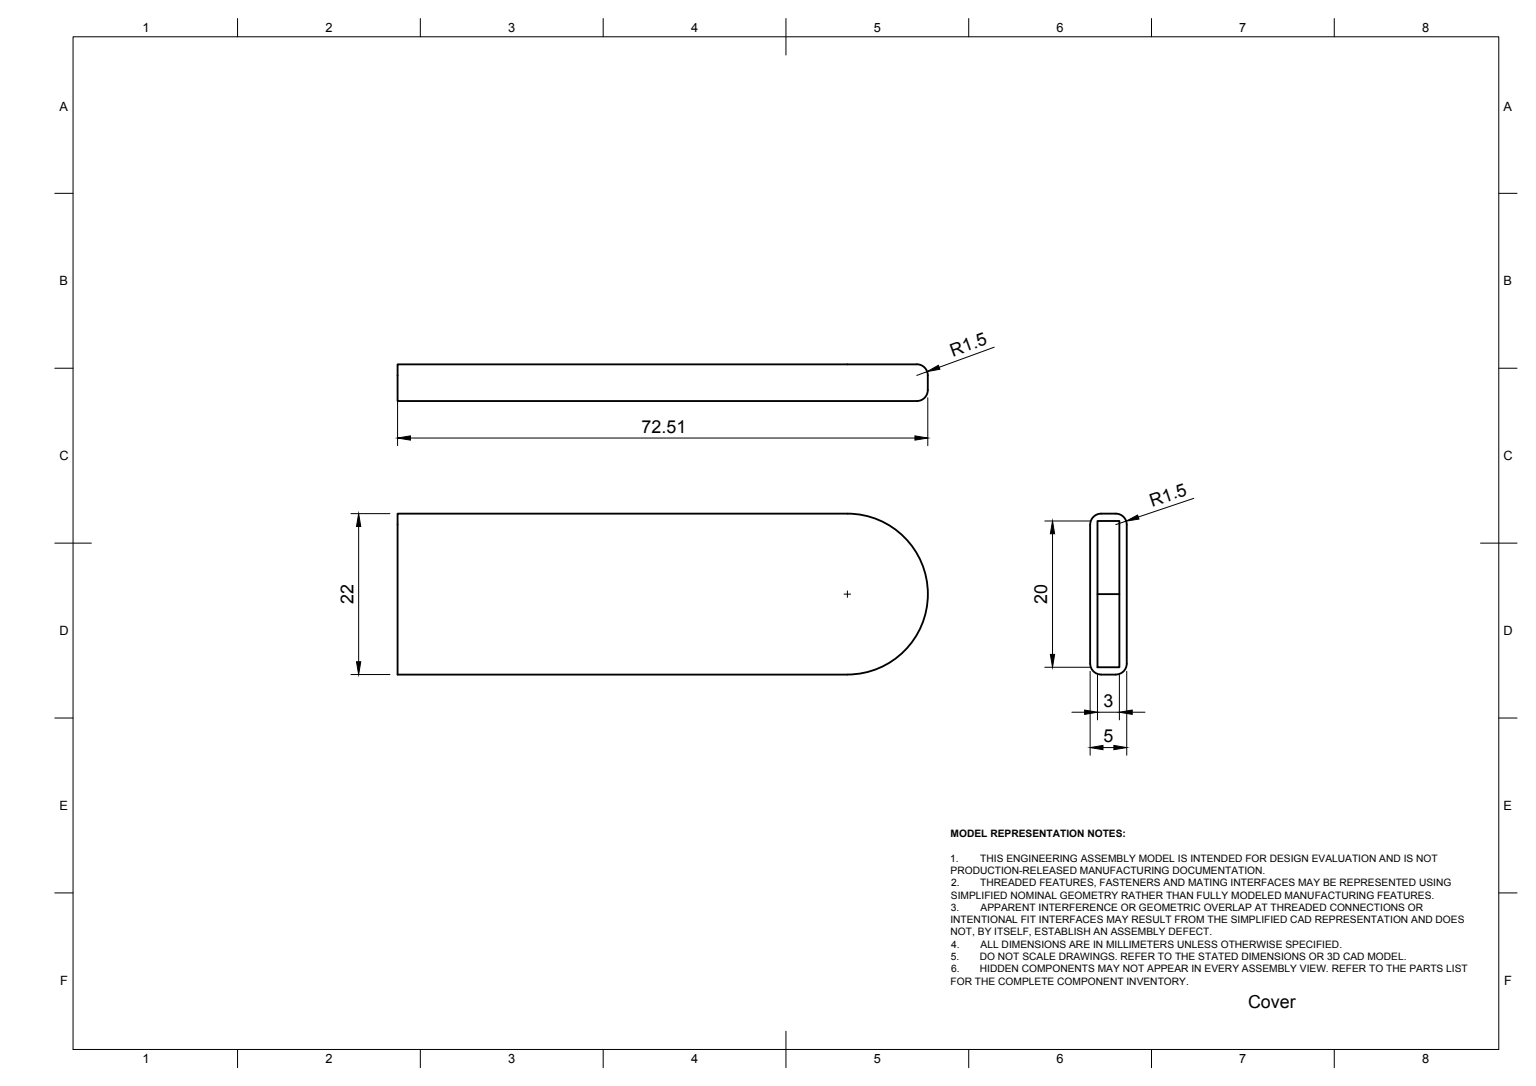
ISO-10303-21;
HEADER;
/* Generated by software containing ST-Developer
 * from STEP Tools, Inc. (www.steptools.com) 
 */

FILE_DESCRIPTION(
/* description */ (''),
/* implementation_level */ '2;1');

FILE_NAME(
/* name */ 'Cover.step',
/* time_stamp */ '2026-10-06T12:47:13-07:00',
/* author */ (''),
/* organization */ (''),
/* preprocessor_version */ 'ST-DEVELOPER v20.2',
/* originating_system */ 'Autodesk Translation Framework v15.15.0.0',
/* authorisation */ '');

FILE_SCHEMA (('AUTOMOTIVE_DESIGN { 1 0 10303 214 3 1 1 }'));
ENDSEC;

DATA;
#10=MECHANICAL_DESIGN_GEOMETRIC_PRESENTATION_REPRESENTATION('',(#68),#42667);
#50=SHAPE_REPRESENTATION_RELATIONSHIP('SRR','None',#42703,#59);
#59=ADVANCED_BREP_SHAPE_REPRESENTATION('',(#77),#42659);
#68=STYLED_ITEM('',(#42756),#77);
#77=MANIFOLD_SOLID_BREP('Body1',#4033);
#387=FACE_BOUND('',#884,.T.);
#403=CYLINDRICAL_SURFACE('',#4197,1.5);
#404=CYLINDRICAL_SURFACE('',#4204,1.5);
#405=CYLINDRICAL_SURFACE('',#4207,11.);
#406=CYLINDRICAL_SURFACE('',#4210,1.5);
#407=CYLINDRICAL_SURFACE('',#4216,1.5);
#408=CYLINDRICAL_SURFACE('',#4220,30.);
#409=CYLINDRICAL_SURFACE('',#4224,30.);
#503=TOROIDAL_SURFACE('',#4200,9.5,1.5);
#504=TOROIDAL_SURFACE('',#4213,9.5,1.5);
#544=CIRCLE('',#4198,1.5);
#545=CIRCLE('',#4199,1.5);
#546=CIRCLE('',#4201,1.5);
#547=CIRCLE('',#4202,11.);
#548=CIRCLE('',#4203,9.5);
#549=CIRCLE('',#4205,1.5);
#550=CIRCLE('',#4208,11.);
#551=CIRCLE('',#4211,1.5);
#552=CIRCLE('',#4212,1.5);
#553=CIRCLE('',#4214,1.5);
#554=CIRCLE('',#4215,9.5);
#555=CIRCLE('',#4217,1.5);
#556=CIRCLE('',#4221,30.);
#557=CIRCLE('',#4222,30.);
#558=CIRCLE('',#4225,30.);
#559=CIRCLE('',#4226,30.);
#667=FACE_OUTER_BOUND('',#873,.T.);
#668=FACE_OUTER_BOUND('',#874,.T.);
#669=FACE_OUTER_BOUND('',#875,.T.);
#670=FACE_OUTER_BOUND('',#876,.T.);
#671=FACE_OUTER_BOUND('',#877,.T.);
#672=FACE_OUTER_BOUND('',#878,.T.);
#673=FACE_OUTER_BOUND('',#879,.T.);
#674=FACE_OUTER_BOUND('',#880,.T.);
#675=FACE_OUTER_BOUND('',#881,.T.);
#676=FACE_OUTER_BOUND('',#882,.T.);
#677=FACE_OUTER_BOUND('',#883,.T.);
#678=FACE_OUTER_BOUND('',#885,.T.);
#679=FACE_OUTER_BOUND('',#886,.T.);
#680=FACE_OUTER_BOUND('',#887,.T.);
#681=FACE_OUTER_BOUND('',#888,.T.);
#682=FACE_OUTER_BOUND('',#889,.T.);
#683=FACE_OUTER_BOUND('',#890,.T.);
#684=FACE_OUTER_BOUND('',#891,.T.);
#873=EDGE_LOOP('',(#2660,#2661,#2662,#2663));
#874=EDGE_LOOP('',(#2664,#2665,#2666,#2667));
#875=EDGE_LOOP('',(#2668,#2669,#2670,#2671));
#876=EDGE_LOOP('',(#2672,#2673,#2674,#2675));
#877=EDGE_LOOP('',(#2676,#2677,#2678,#2679));
#878=EDGE_LOOP('',(#2680,#2681,#2682,#2683));
#879=EDGE_LOOP('',(#2684,#2685,#2686,#2687));
#880=EDGE_LOOP('',(#2688,#2689,#2690,#2691));
#881=EDGE_LOOP('',(#2692,#2693,#2694,#2695));
#882=EDGE_LOOP('',(#2696,#2697,#2698,#2699));
#883=EDGE_LOOP('',(#2700,#2701,#2702,#2703,#2704,#2705,#2706,#2707));
#884=EDGE_LOOP('',(#2708,#2709,#2710,#2711));
#885=EDGE_LOOP('',(#2712,#2713,#2714,#2715));
#886=EDGE_LOOP('',(#2716,#2717,#2718,#2719));
#887=EDGE_LOOP('',(#2720,#2721,#2722,#2723));
#888=EDGE_LOOP('',(#2724,#2725,#2726,#2727,#2728));
#889=EDGE_LOOP('',(#2729,#2730,#2731,#2732));
#890=EDGE_LOOP('',(#2733,#2734,#2735,#2736,#2737));
#891=EDGE_LOOP('',(#2738,#2739,#2740,#2741));
#1082=LINE('',#5866,#1295);
#1083=LINE('',#5869,#1296);
#1084=LINE('',#5880,#1297);
#1085=LINE('',#5881,#1298);
#1086=LINE('',#5884,#1299);
#1087=LINE('',#5886,#1300);
#1088=LINE('',#5887,#1301);
#1089=LINE('',#5890,#1302);
#1090=LINE('',#5894,#1303);
#1091=LINE('',#5895,#1304);
#1092=LINE('',#5900,#1305);
#1093=LINE('',#5909,#1306);
#1094=LINE('',#5911,#1307);
#1095=LINE('',#5913,#1308);
#1096=LINE('',#5916,#1309);
#1097=LINE('',#5918,#1310);
#1098=LINE('',#5920,#1311);
#1099=LINE('',#5921,#1312);
#1100=LINE('',#5927,#1313);
#1101=LINE('',#5930,#1314);
#1102=LINE('',#5932,#1315);
#1103=LINE('',#5933,#1316);
#1104=LINE('',#5938,#1317);
#1105=LINE('',#5941,#1318);
#1106=LINE('',#5943,#1319);
#1295=VECTOR('',#4615,10.);
#1296=VECTOR('',#4618,10.);
#1297=VECTOR('',#4631,10.);
#1298=VECTOR('',#4632,10.);
#1299=VECTOR('',#4635,10.);
#1300=VECTOR('',#4636,10.);
#1301=VECTOR('',#4637,10.);
#1302=VECTOR('',#4640,10.);
#1303=VECTOR('',#4645,10.);
#1304=VECTOR('',#4646,10.);
#1305=VECTOR('',#4651,10.);
#1306=VECTOR('',#4664,10.);
#1307=VECTOR('',#4667,10.);
#1308=VECTOR('',#4670,10.);
#1309=VECTOR('',#4671,10.);
#1310=VECTOR('',#4672,10.);
#1311=VECTOR('',#4673,10.);
#1312=VECTOR('',#4674,10.);
#1313=VECTOR('',#4679,10.);
#1314=VECTOR('',#4682,30.);
#1315=VECTOR('',#4685,10.);
#1316=VECTOR('',#4686,10.);
#1317=VECTOR('',#4691,30.);
#1318=VECTOR('',#4696,10.);
#1319=VECTOR('',#4699,10.);
#1516=VERTEX_POINT('',#5862);
#1517=VERTEX_POINT('',#5863);
#1518=VERTEX_POINT('',#5865);
#1519=VERTEX_POINT('',#5867);
#1520=VERTEX_POINT('',#5871);
#1521=VERTEX_POINT('',#5872);
#1522=VERTEX_POINT('',#5877);
#1523=VERTEX_POINT('',#5878);
#1524=VERTEX_POINT('',#5883);
#1525=VERTEX_POINT('',#5885);
#1526=VERTEX_POINT('',#5889);
#1527=VERTEX_POINT('',#5893);
#1528=VERTEX_POINT('',#5897);
#1529=VERTEX_POINT('',#5899);
#1530=VERTEX_POINT('',#5903);
#1531=VERTEX_POINT('',#5907);
#1532=VERTEX_POINT('',#5914);
#1533=VERTEX_POINT('',#5915);
#1534=VERTEX_POINT('',#5917);
#1535=VERTEX_POINT('',#5919);
#1536=VERTEX_POINT('',#5923);
#1537=VERTEX_POINT('',#5924);
#1538=VERTEX_POINT('',#5926);
#1539=VERTEX_POINT('',#5928);
#1540=VERTEX_POINT('',#5935);
#1541=VERTEX_POINT('',#5937);
#1981=EDGE_CURVE('',#1516,#1517,#544,.T.);
#1982=EDGE_CURVE('',#1517,#1518,#1082,.T.);
#1983=EDGE_CURVE('',#1518,#1519,#545,.T.);
#1984=EDGE_CURVE('',#1519,#1516,#1083,.T.);
#1985=EDGE_CURVE('',#1520,#1521,#546,.T.);
#1986=EDGE_CURVE('',#1521,#1519,#547,.T.);
#1987=EDGE_CURVE('',#1518,#1520,#548,.T.);
#1988=EDGE_CURVE('',#1522,#1523,#549,.T.);
#1989=EDGE_CURVE('',#1523,#1521,#1084,.T.);
#1990=EDGE_CURVE('',#1520,#1522,#1085,.T.);
#1991=EDGE_CURVE('',#1519,#1524,#1086,.T.);
#1992=EDGE_CURVE('',#1525,#1524,#1087,.T.);
#1993=EDGE_CURVE('',#1516,#1525,#1088,.T.);
#1994=EDGE_CURVE('',#1521,#1526,#1089,.T.);
#1995=EDGE_CURVE('',#1524,#1526,#550,.T.);
#1996=EDGE_CURVE('',#1523,#1527,#1090,.T.);
#1997=EDGE_CURVE('',#1526,#1527,#1091,.T.);
#1998=EDGE_CURVE('',#1527,#1528,#551,.T.);
#1999=EDGE_CURVE('',#1528,#1529,#1092,.T.);
#2000=EDGE_CURVE('',#1529,#1526,#552,.T.);
#2001=EDGE_CURVE('',#1530,#1524,#553,.T.);
#2002=EDGE_CURVE('',#1529,#1530,#554,.T.);
#2003=EDGE_CURVE('',#1531,#1525,#555,.T.);
#2004=EDGE_CURVE('',#1530,#1531,#1093,.T.);
#2005=EDGE_CURVE('',#1531,#1528,#1094,.T.);
#2006=EDGE_CURVE('',#1517,#1522,#1095,.T.);
#2007=EDGE_CURVE('',#1532,#1533,#1096,.T.);
#2008=EDGE_CURVE('',#1534,#1533,#1097,.T.);
#2009=EDGE_CURVE('',#1535,#1534,#1098,.T.);
#2010=EDGE_CURVE('',#1535,#1532,#1099,.T.);
#2011=EDGE_CURVE('',#1536,#1537,#556,.T.);
#2012=EDGE_CURVE('',#1537,#1538,#1100,.T.);
#2013=EDGE_CURVE('',#1538,#1539,#557,.T.);
#2014=EDGE_CURVE('',#1536,#1539,#1101,.T.);
#2015=EDGE_CURVE('',#1539,#1532,#1102,.T.);
#2016=EDGE_CURVE('',#1535,#1536,#1103,.T.);
#2017=EDGE_CURVE('',#1540,#1537,#558,.T.);
#2018=EDGE_CURVE('',#1540,#1541,#1104,.T.);
#2019=EDGE_CURVE('',#1538,#1541,#559,.T.);
#2020=EDGE_CURVE('',#1534,#1540,#1105,.T.);
#2021=EDGE_CURVE('',#1541,#1533,#1106,.T.);
#2660=ORIENTED_EDGE('',*,*,#1981,.T.);
#2661=ORIENTED_EDGE('',*,*,#1982,.T.);
#2662=ORIENTED_EDGE('',*,*,#1983,.T.);
#2663=ORIENTED_EDGE('',*,*,#1984,.T.);
#2664=ORIENTED_EDGE('',*,*,#1985,.T.);
#2665=ORIENTED_EDGE('',*,*,#1986,.T.);
#2666=ORIENTED_EDGE('',*,*,#1983,.F.);
#2667=ORIENTED_EDGE('',*,*,#1987,.T.);
#2668=ORIENTED_EDGE('',*,*,#1988,.T.);
#2669=ORIENTED_EDGE('',*,*,#1989,.T.);
#2670=ORIENTED_EDGE('',*,*,#1985,.F.);
#2671=ORIENTED_EDGE('',*,*,#1990,.T.);
#2672=ORIENTED_EDGE('',*,*,#1984,.F.);
#2673=ORIENTED_EDGE('',*,*,#1991,.T.);
#2674=ORIENTED_EDGE('',*,*,#1992,.F.);
#2675=ORIENTED_EDGE('',*,*,#1993,.F.);
#2676=ORIENTED_EDGE('',*,*,#1986,.F.);
#2677=ORIENTED_EDGE('',*,*,#1994,.T.);
#2678=ORIENTED_EDGE('',*,*,#1995,.F.);
#2679=ORIENTED_EDGE('',*,*,#1991,.F.);
#2680=ORIENTED_EDGE('',*,*,#1989,.F.);
#2681=ORIENTED_EDGE('',*,*,#1996,.T.);
#2682=ORIENTED_EDGE('',*,*,#1997,.F.);
#2683=ORIENTED_EDGE('',*,*,#1994,.F.);
#2684=ORIENTED_EDGE('',*,*,#1998,.T.);
#2685=ORIENTED_EDGE('',*,*,#1999,.T.);
#2686=ORIENTED_EDGE('',*,*,#2000,.T.);
#2687=ORIENTED_EDGE('',*,*,#1997,.T.);
#2688=ORIENTED_EDGE('',*,*,#2001,.T.);
#2689=ORIENTED_EDGE('',*,*,#1995,.T.);
#2690=ORIENTED_EDGE('',*,*,#2000,.F.);
#2691=ORIENTED_EDGE('',*,*,#2002,.T.);
#2692=ORIENTED_EDGE('',*,*,#2003,.T.);
#2693=ORIENTED_EDGE('',*,*,#1992,.T.);
#2694=ORIENTED_EDGE('',*,*,#2001,.F.);
#2695=ORIENTED_EDGE('',*,*,#2004,.T.);
#2696=ORIENTED_EDGE('',*,*,#2004,.F.);
#2697=ORIENTED_EDGE('',*,*,#2002,.F.);
#2698=ORIENTED_EDGE('',*,*,#1999,.F.);
#2699=ORIENTED_EDGE('',*,*,#2005,.F.);
#2700=ORIENTED_EDGE('',*,*,#1981,.F.);
#2701=ORIENTED_EDGE('',*,*,#1993,.T.);
#2702=ORIENTED_EDGE('',*,*,#2003,.F.);
#2703=ORIENTED_EDGE('',*,*,#2005,.T.);
#2704=ORIENTED_EDGE('',*,*,#1998,.F.);
#2705=ORIENTED_EDGE('',*,*,#1996,.F.);
#2706=ORIENTED_EDGE('',*,*,#1988,.F.);
#2707=ORIENTED_EDGE('',*,*,#2006,.F.);
#2708=ORIENTED_EDGE('',*,*,#2007,.T.);
#2709=ORIENTED_EDGE('',*,*,#2008,.F.);
#2710=ORIENTED_EDGE('',*,*,#2009,.F.);
#2711=ORIENTED_EDGE('',*,*,#2010,.T.);
#2712=ORIENTED_EDGE('',*,*,#2011,.T.);
#2713=ORIENTED_EDGE('',*,*,#2012,.T.);
#2714=ORIENTED_EDGE('',*,*,#2013,.T.);
#2715=ORIENTED_EDGE('',*,*,#2014,.F.);
#2716=ORIENTED_EDGE('',*,*,#2014,.T.);
#2717=ORIENTED_EDGE('',*,*,#2015,.T.);
#2718=ORIENTED_EDGE('',*,*,#2010,.F.);
#2719=ORIENTED_EDGE('',*,*,#2016,.T.);
#2720=ORIENTED_EDGE('',*,*,#2017,.F.);
#2721=ORIENTED_EDGE('',*,*,#2018,.T.);
#2722=ORIENTED_EDGE('',*,*,#2019,.F.);
#2723=ORIENTED_EDGE('',*,*,#2012,.F.);
#2724=ORIENTED_EDGE('',*,*,#2017,.T.);
#2725=ORIENTED_EDGE('',*,*,#2011,.F.);
#2726=ORIENTED_EDGE('',*,*,#2016,.F.);
#2727=ORIENTED_EDGE('',*,*,#2009,.T.);
#2728=ORIENTED_EDGE('',*,*,#2020,.T.);
#2729=ORIENTED_EDGE('',*,*,#2018,.F.);
#2730=ORIENTED_EDGE('',*,*,#2020,.F.);
#2731=ORIENTED_EDGE('',*,*,#2008,.T.);
#2732=ORIENTED_EDGE('',*,*,#2021,.F.);
#2733=ORIENTED_EDGE('',*,*,#2019,.T.);
#2734=ORIENTED_EDGE('',*,*,#2021,.T.);
#2735=ORIENTED_EDGE('',*,*,#2007,.F.);
#2736=ORIENTED_EDGE('',*,*,#2015,.F.);
#2737=ORIENTED_EDGE('',*,*,#2013,.F.);
#2738=ORIENTED_EDGE('',*,*,#1982,.F.);
#2739=ORIENTED_EDGE('',*,*,#2006,.T.);
#2740=ORIENTED_EDGE('',*,*,#1990,.F.);
#2741=ORIENTED_EDGE('',*,*,#1987,.F.);
#3788=PLANE('',#4206);
#3789=PLANE('',#4209);
#3790=PLANE('',#4218);
#3791=PLANE('',#4219);
#3792=PLANE('',#4223);
#3793=PLANE('',#4227);
#3794=PLANE('',#4228);
#3795=PLANE('',#4229);
#3796=PLANE('',#4230);
#3863=ADVANCED_FACE('',(#667),#403,.T.);
#3864=ADVANCED_FACE('',(#668),#503,.T.);
#3865=ADVANCED_FACE('',(#669),#404,.T.);
#3866=ADVANCED_FACE('',(#670),#3788,.F.);
#3867=ADVANCED_FACE('',(#671),#405,.T.);
#3868=ADVANCED_FACE('',(#672),#3789,.T.);
#3869=ADVANCED_FACE('',(#673),#406,.T.);
#3870=ADVANCED_FACE('',(#674),#504,.T.);
#3871=ADVANCED_FACE('',(#675),#407,.T.);
#3872=ADVANCED_FACE('',(#676),#3790,.T.);
#3873=ADVANCED_FACE('',(#677,#387),#3791,.T.);
#3874=ADVANCED_FACE('',(#678),#408,.F.);
#3875=ADVANCED_FACE('',(#679),#3792,.F.);
#3876=ADVANCED_FACE('',(#680),#409,.F.);
#3877=ADVANCED_FACE('',(#681),#3793,.T.);
#3878=ADVANCED_FACE('',(#682),#3794,.T.);
#3879=ADVANCED_FACE('',(#683),#3795,.T.);
#3880=ADVANCED_FACE('',(#684),#3796,.T.);
#4033=CLOSED_SHELL('',(#3863,#3864,#3865,#3866,#3867,#3868,#3869,#3870,
#3871,#3872,#3873,#3874,#3875,#3876,#3877,#3878,#3879,#3880));
#4196=AXIS2_PLACEMENT_3D('',#5860,#4609,#4610);
#4197=AXIS2_PLACEMENT_3D('',#5861,#4611,#4612);
#4198=AXIS2_PLACEMENT_3D('',#5864,#4613,#4614);
#4199=AXIS2_PLACEMENT_3D('',#5868,#4616,#4617);
#4200=AXIS2_PLACEMENT_3D('',#5870,#4619,#4620);
#4201=AXIS2_PLACEMENT_3D('',#5873,#4621,#4622);
#4202=AXIS2_PLACEMENT_3D('',#5874,#4623,#4624);
#4203=AXIS2_PLACEMENT_3D('',#5875,#4625,#4626);
#4204=AXIS2_PLACEMENT_3D('',#5876,#4627,#4628);
#4205=AXIS2_PLACEMENT_3D('',#5879,#4629,#4630);
#4206=AXIS2_PLACEMENT_3D('',#5882,#4633,#4634);
#4207=AXIS2_PLACEMENT_3D('',#5888,#4638,#4639);
#4208=AXIS2_PLACEMENT_3D('',#5891,#4641,#4642);
#4209=AXIS2_PLACEMENT_3D('',#5892,#4643,#4644);
#4210=AXIS2_PLACEMENT_3D('',#5896,#4647,#4648);
#4211=AXIS2_PLACEMENT_3D('',#5898,#4649,#4650);
#4212=AXIS2_PLACEMENT_3D('',#5901,#4652,#4653);
#4213=AXIS2_PLACEMENT_3D('',#5902,#4654,#4655);
#4214=AXIS2_PLACEMENT_3D('',#5904,#4656,#4657);
#4215=AXIS2_PLACEMENT_3D('',#5905,#4658,#4659);
#4216=AXIS2_PLACEMENT_3D('',#5906,#4660,#4661);
#4217=AXIS2_PLACEMENT_3D('',#5908,#4662,#4663);
#4218=AXIS2_PLACEMENT_3D('',#5910,#4665,#4666);
#4219=AXIS2_PLACEMENT_3D('',#5912,#4668,#4669);
#4220=AXIS2_PLACEMENT_3D('',#5922,#4675,#4676);
#4221=AXIS2_PLACEMENT_3D('',#5925,#4677,#4678);
#4222=AXIS2_PLACEMENT_3D('',#5929,#4680,#4681);
#4223=AXIS2_PLACEMENT_3D('',#5931,#4683,#4684);
#4224=AXIS2_PLACEMENT_3D('',#5934,#4687,#4688);
#4225=AXIS2_PLACEMENT_3D('',#5936,#4689,#4690);
#4226=AXIS2_PLACEMENT_3D('',#5939,#4692,#4693);
#4227=AXIS2_PLACEMENT_3D('',#5940,#4694,#4695);
#4228=AXIS2_PLACEMENT_3D('',#5942,#4697,#4698);
#4229=AXIS2_PLACEMENT_3D('',#5944,#4700,#4701);
#4230=AXIS2_PLACEMENT_3D('',#5945,#4702,#4703);
#4609=DIRECTION('axis',(0.,0.,1.));
#4610=DIRECTION('refdir',(1.,0.,0.));
#4611=DIRECTION('center_axis',(0.,1.,0.));
#4612=DIRECTION('ref_axis',(-0.707106781186547,0.,-0.707106781186548));
#4613=DIRECTION('center_axis',(0.,-1.,0.));
#4614=DIRECTION('ref_axis',(-0.707106781186547,0.,-0.707106781186548));
#4615=DIRECTION('',(0.,-1.,0.));
#4616=DIRECTION('center_axis',(0.,1.,0.));
#4617=DIRECTION('ref_axis',(0.,0.,-1.));
#4618=DIRECTION('',(0.,1.,0.));
#4619=DIRECTION('center_axis',(0.,0.,1.));
#4620=DIRECTION('ref_axis',(1.,0.,0.));
#4621=DIRECTION('center_axis',(0.,-1.,0.));
#4622=DIRECTION('ref_axis',(0.,0.,-1.));
#4623=DIRECTION('center_axis',(0.,0.,-1.));
#4624=DIRECTION('ref_axis',(1.00929365875014E-16,-1.,0.));
#4625=DIRECTION('center_axis',(0.,0.,1.));
#4626=DIRECTION('ref_axis',(1.00929365875014E-16,-1.,0.));
#4627=DIRECTION('center_axis',(0.,1.,0.));
#4628=DIRECTION('ref_axis',(0.707106781186547,0.,-0.707106781186548));
#4629=DIRECTION('center_axis',(0.,-1.,0.));
#4630=DIRECTION('ref_axis',(0.707106781186547,0.,-0.707106781186548));
#4631=DIRECTION('',(0.,-1.,0.));
#4632=DIRECTION('',(0.,1.,0.));
#4633=DIRECTION('center_axis',(1.,0.,0.));
#4634=DIRECTION('ref_axis',(0.,0.,-1.));
#4635=DIRECTION('',(0.,0.,1.));
#4636=DIRECTION('',(0.,-1.,0.));
#4637=DIRECTION('',(0.,0.,1.));
#4638=DIRECTION('center_axis',(0.,0.,-1.));
#4639=DIRECTION('ref_axis',(0.707106781186547,-0.707106781186548,0.));
#4640=DIRECTION('',(0.,0.,1.));
#4641=DIRECTION('center_axis',(0.,0.,1.));
#4642=DIRECTION('ref_axis',(-5.04646829375071E-16,-1.,0.));
#4643=DIRECTION('center_axis',(1.,0.,0.));
#4644=DIRECTION('ref_axis',(0.,0.,-1.));
#4645=DIRECTION('',(0.,0.,1.));
#4646=DIRECTION('',(0.,1.,0.));
#4647=DIRECTION('center_axis',(0.,-1.,0.));
#4648=DIRECTION('ref_axis',(0.707106781186547,0.,0.707106781186548));
#4649=DIRECTION('center_axis',(0.,-1.,0.));
#4650=DIRECTION('ref_axis',(0.707106781186547,0.,0.707106781186548));
#4651=DIRECTION('',(0.,-1.,0.));
#4652=DIRECTION('center_axis',(0.,1.,0.));
#4653=DIRECTION('ref_axis',(0.,0.,1.));
#4654=DIRECTION('center_axis',(0.,0.,1.));
#4655=DIRECTION('ref_axis',(1.,0.,0.));
#4656=DIRECTION('center_axis',(0.,-1.,0.));
#4657=DIRECTION('ref_axis',(0.,0.,1.));
#4658=DIRECTION('center_axis',(0.,0.,-1.));
#4659=DIRECTION('ref_axis',(-5.04646829375071E-16,-1.,0.));
#4660=DIRECTION('center_axis',(0.,-1.,0.));
#4661=DIRECTION('ref_axis',(-0.707106781186543,0.,0.707106781186552));
#4662=DIRECTION('center_axis',(0.,-1.,0.));
#4663=DIRECTION('ref_axis',(-0.707106781186543,0.,0.707106781186552));
#4664=DIRECTION('',(0.,1.,0.));
#4665=DIRECTION('center_axis',(0.,0.,1.));
#4666=DIRECTION('ref_axis',(0.,-1.,0.));
#4667=DIRECTION('',(1.,0.,0.));
#4668=DIRECTION('center_axis',(0.,1.,0.));
#4669=DIRECTION('ref_axis',(0.,0.,1.));
#4670=DIRECTION('',(1.,0.,0.));
#4671=DIRECTION('',(1.,0.,0.));
#4672=DIRECTION('',(0.,0.,-1.));
#4673=DIRECTION('',(1.,0.,0.));
#4674=DIRECTION('',(0.,0.,-1.));
#4675=DIRECTION('center_axis',(0.,0.,-1.));
#4676=DIRECTION('ref_axis',(-0.666666666666667,-0.74535599249993,0.));
#4677=DIRECTION('center_axis',(0.,0.,1.));
#4678=DIRECTION('ref_axis',(-0.666666666666667,-0.74535599249993,0.));
#4679=DIRECTION('',(0.,0.,-1.));
#4680=DIRECTION('center_axis',(0.,0.,-1.));
#4681=DIRECTION('ref_axis',(-0.666666666666667,-0.74535599249993,0.));
#4682=DIRECTION('',(0.,0.,-1.));
#4683=DIRECTION('center_axis',(-1.,0.,0.));
#4684=DIRECTION('ref_axis',(0.,0.,1.));
#4685=DIRECTION('',(0.,1.,0.));
#4686=DIRECTION('',(0.,-1.,0.));
#4687=DIRECTION('center_axis',(0.,0.,1.));
#4688=DIRECTION('ref_axis',(0.666666666666667,-0.74535599249993,0.));
#4689=DIRECTION('center_axis',(0.,0.,-1.));
#4690=DIRECTION('ref_axis',(0.666666666666667,-0.74535599249993,0.));
#4691=DIRECTION('',(0.,0.,-1.));
#4692=DIRECTION('center_axis',(0.,0.,1.));
#4693=DIRECTION('ref_axis',(0.666666666666667,-0.74535599249993,0.));
#4694=DIRECTION('center_axis',(0.,0.,-1.));
#4695=DIRECTION('ref_axis',(0.,1.,0.));
#4696=DIRECTION('',(0.,-1.,0.));
#4697=DIRECTION('center_axis',(-1.,0.,0.));
#4698=DIRECTION('ref_axis',(0.,0.,1.));
#4699=DIRECTION('',(0.,1.,0.));
#4700=DIRECTION('center_axis',(0.,0.,1.));
#4701=DIRECTION('ref_axis',(0.,-1.,0.));
#4702=DIRECTION('center_axis',(0.,0.,-1.));
#4703=DIRECTION('ref_axis',(0.,1.,0.));
#5860=CARTESIAN_POINT('',(0.,0.,0.));
#5861=CARTESIAN_POINT('Origin',(-9.5,-85.5138405476197,49.642135623731));
#5862=CARTESIAN_POINT('',(-11.,-31.1289553192861,49.642135623731));
#5863=CARTESIAN_POINT('',(-9.5,-31.1289553192861,48.142135623731));
#5864=CARTESIAN_POINT('Origin',(-9.5,-31.1289553192861,49.642135623731));
#5865=CARTESIAN_POINT('',(-9.5,-92.6421356237309,48.142135623731));
#5866=CARTESIAN_POINT('',(-9.5,-85.5138405476197,48.142135623731));
#5867=CARTESIAN_POINT('',(-11.,-92.6421356237309,49.642135623731));
#5868=CARTESIAN_POINT('Origin',(-9.5,-92.6421356237309,49.642135623731));
#5869=CARTESIAN_POINT('',(-11.,-85.5138405476197,49.642135623731));
#5870=CARTESIAN_POINT('Origin',(0.,-92.6421356237309,49.642135623731));
#5871=CARTESIAN_POINT('',(9.5,-92.6421356237309,48.142135623731));
#5872=CARTESIAN_POINT('',(11.,-92.6421356237309,49.642135623731));
#5873=CARTESIAN_POINT('Origin',(9.5,-92.6421356237309,49.642135623731));
#5874=CARTESIAN_POINT('Origin',(0.,-92.6421356237309,49.642135623731));
#5875=CARTESIAN_POINT('Origin',(0.,-92.6421356237309,48.142135623731));
#5876=CARTESIAN_POINT('Origin',(9.5,-85.5138405476197,49.642135623731));
#5877=CARTESIAN_POINT('',(9.5,-31.1289553192861,48.142135623731));
#5878=CARTESIAN_POINT('',(11.,-31.1289553192861,49.642135623731));
#5879=CARTESIAN_POINT('Origin',(9.5,-31.1289553192861,49.642135623731));
#5880=CARTESIAN_POINT('',(11.,-85.5138405476197,49.642135623731));
#5881=CARTESIAN_POINT('',(9.5,-85.5138405476197,48.142135623731));
#5882=CARTESIAN_POINT('Origin',(-11.,-67.3855454715085,50.642135623731));
#5883=CARTESIAN_POINT('',(-11.,-92.6421356237309,51.642135623731));
#5884=CARTESIAN_POINT('',(-11.,-92.6421356237309,51.892135623731));
#5885=CARTESIAN_POINT('',(-11.,-31.1289553192861,51.6421356237309));
#5886=CARTESIAN_POINT('',(-11.,-49.2572503953973,51.6421356237309));
#5887=CARTESIAN_POINT('',(-11.,-31.1289553192861,53.142135623731));
#5888=CARTESIAN_POINT('Origin',(0.,-92.6421356237309,51.892135623731));
#5889=CARTESIAN_POINT('',(11.,-92.6421356237309,51.642135623731));
#5890=CARTESIAN_POINT('',(11.,-92.6421356237309,51.892135623731));
#5891=CARTESIAN_POINT('Origin',(0.,-92.6421356237309,51.642135623731));
#5892=CARTESIAN_POINT('Origin',(11.,-67.3855454715085,50.642135623731));
#5893=CARTESIAN_POINT('',(11.,-31.1289553192861,51.642135623731));
#5894=CARTESIAN_POINT('',(11.,-31.1289553192861,53.142135623731));
#5895=CARTESIAN_POINT('',(11.,-49.2572503953973,51.642135623731));
#5896=CARTESIAN_POINT('Origin',(9.5,-49.2572503953973,51.642135623731));
#5897=CARTESIAN_POINT('',(9.5,-31.1289553192861,53.142135623731));
#5898=CARTESIAN_POINT('Origin',(9.5,-31.1289553192861,51.642135623731));
#5899=CARTESIAN_POINT('',(9.5,-92.6421356237309,53.142135623731));
#5900=CARTESIAN_POINT('',(9.5,-49.2572503953973,53.142135623731));
#5901=CARTESIAN_POINT('Origin',(9.5,-92.6421356237309,51.642135623731));
#5902=CARTESIAN_POINT('Origin',(0.,-92.6421356237309,51.642135623731));
#5903=CARTESIAN_POINT('',(-9.5,-92.6421356237309,53.142135623731));
#5904=CARTESIAN_POINT('Origin',(-9.5,-92.6421356237309,51.642135623731));
#5905=CARTESIAN_POINT('Origin',(0.,-92.6421356237309,53.142135623731));
#5906=CARTESIAN_POINT('Origin',(-9.5,-49.2572503953973,51.6421356237309));
#5907=CARTESIAN_POINT('',(-9.5,-31.1289553192861,53.142135623731));
#5908=CARTESIAN_POINT('Origin',(-9.5,-31.1289553192861,51.6421356237309));
#5909=CARTESIAN_POINT('',(-9.5,-49.2572503953973,53.142135623731));
#5910=CARTESIAN_POINT('Origin',(0.,-31.1289553192861,53.142135623731));
#5911=CARTESIAN_POINT('',(0.,-31.1289553192861,53.142135623731));
#5912=CARTESIAN_POINT('Origin',(0.,-31.1289553192861,52.142135623731));
#5913=CARTESIAN_POINT('',(0.,-31.1289553192861,48.142135623731));
#5914=CARTESIAN_POINT('',(-10.,-31.1289553192861,49.142135623731));
#5915=CARTESIAN_POINT('',(10.,-31.1289553192861,49.142135623731));
#5916=CARTESIAN_POINT('',(0.,-31.1289553192861,49.142135623731));
#5917=CARTESIAN_POINT('',(10.,-31.1289553192861,52.142135623731));
#5918=CARTESIAN_POINT('',(10.,-31.1289553192861,53.142135623731));
#5919=CARTESIAN_POINT('',(-10.,-31.1289553192861,52.142135623731));
#5920=CARTESIAN_POINT('',(0.,-31.1289553192861,52.142135623731));
#5921=CARTESIAN_POINT('',(-10.,-31.1289553192861,53.142135623731));
#5922=CARTESIAN_POINT('Origin',(20.,-80.281455848733,52.142135623731));
#5923=CARTESIAN_POINT('',(-10.,-80.281455848733,52.142135623731));
#5924=CARTESIAN_POINT('',(0.,-102.642135623731,52.142135623731));
#5925=CARTESIAN_POINT('Origin',(20.,-80.281455848733,52.142135623731));
#5926=CARTESIAN_POINT('',(0.,-102.642135623731,49.142135623731));
#5927=CARTESIAN_POINT('',(0.,-102.642135623731,52.142135623731));
#5928=CARTESIAN_POINT('',(-10.,-80.281455848733,49.142135623731));
#5929=CARTESIAN_POINT('Origin',(20.,-80.281455848733,49.142135623731));
#5930=CARTESIAN_POINT('',(-10.,-80.281455848733,52.142135623731));
#5931=CARTESIAN_POINT('Origin',(-10.,-67.3855454715085,50.642135623731));
#5932=CARTESIAN_POINT('',(-10.,-49.2572503953973,49.142135623731));
#5933=CARTESIAN_POINT('',(-10.,-85.0138405476197,52.142135623731));
#5934=CARTESIAN_POINT('Origin',(-20.,-80.281455848733,52.142135623731));
#5935=CARTESIAN_POINT('',(10.,-80.281455848733,52.142135623731));
#5936=CARTESIAN_POINT('Origin',(-20.,-80.281455848733,52.142135623731));
#5937=CARTESIAN_POINT('',(10.,-80.281455848733,49.142135623731));
#5938=CARTESIAN_POINT('',(10.,-80.281455848733,52.142135623731));
#5939=CARTESIAN_POINT('Origin',(-20.,-80.281455848733,49.142135623731));
#5940=CARTESIAN_POINT('Origin',(0.,-102.642135623731,52.142135623731));
#5941=CARTESIAN_POINT('',(10.,-85.0138405476197,52.142135623731));
#5942=CARTESIAN_POINT('Origin',(10.,-67.3855454715085,50.642135623731));
#5943=CARTESIAN_POINT('',(10.,-49.2572503953973,49.142135623731));
#5944=CARTESIAN_POINT('Origin',(0.,-31.1289553192861,49.142135623731));
#5945=CARTESIAN_POINT('Origin',(0.,-103.642135623731,48.142135623731));
#42648=UNCERTAINTY_MEASURE_WITH_UNIT(LENGTH_MEASURE(0.01),#42668,
'DISTANCE_ACCURACY_VALUE',
'Maximum model space distance between geometric entities at asserted c
onnectivities');
#42656=UNCERTAINTY_MEASURE_WITH_UNIT(LENGTH_MEASURE(0.01),#42668,
'DISTANCE_ACCURACY_VALUE',
'Maximum model space distance between geometric entities at asserted c
onnectivities');
#42659=(
GEOMETRIC_REPRESENTATION_CONTEXT(3)
GLOBAL_UNCERTAINTY_ASSIGNED_CONTEXT((#42648))
GLOBAL_UNIT_ASSIGNED_CONTEXT((#42668,#42670,#42671))
REPRESENTATION_CONTEXT('','3D')
);
#42667=(
GEOMETRIC_REPRESENTATION_CONTEXT(3)
GLOBAL_UNCERTAINTY_ASSIGNED_CONTEXT((#42656))
GLOBAL_UNIT_ASSIGNED_CONTEXT((#42668,#42670,#42671))
REPRESENTATION_CONTEXT('','3D')
);
#42668=(
LENGTH_UNIT()
NAMED_UNIT(*)
SI_UNIT(.MILLI.,.METRE.)
);
#42670=(
NAMED_UNIT(*)
PLANE_ANGLE_UNIT()
SI_UNIT($,.RADIAN.)
);
#42671=(
NAMED_UNIT(*)
SI_UNIT($,.STERADIAN.)
SOLID_ANGLE_UNIT()
);
#42674=SHAPE_DEFINITION_REPRESENTATION(#42684,#42703);
#42684=PRODUCT_DEFINITION_SHAPE('',$,#42714);
#42703=SHAPE_REPRESENTATION('',(#4196),#42659);
#42711=PRODUCT_DEFINITION_CONTEXT('part definition',#42743,'design');
#42714=PRODUCT_DEFINITION('Cover','Cover',#42724,#42711);
#42724=PRODUCT_DEFINITION_FORMATION('',$,#42747);
#42743=APPLICATION_CONTEXT(
'Core Data for Automotive Mechanical Design Process');
#42744=PRODUCT_CONTEXT('part definition',#42743,'mechanical');
#42747=PRODUCT('Cover','Cover',$,(#42744));
#42756=PRESENTATION_STYLE_ASSIGNMENT((#42758));
#42758=SURFACE_STYLE_USAGE(.BOTH.,#42760);
#42760=SURFACE_SIDE_STYLE('',(#42762));
#42762=SURFACE_STYLE_FILL_AREA(#42764);
#42764=FILL_AREA_STYLE('Opaque(160,160,160)',(#42766));
#42766=FILL_AREA_STYLE_COLOUR('Opaque(160,160,160)',#42768);
#42768=COLOUR_RGB('Opaque(160,160,160)', 0.09019608, 0.27058824, 0.51372549);
ENDSEC;
END-ISO-10303-21;
